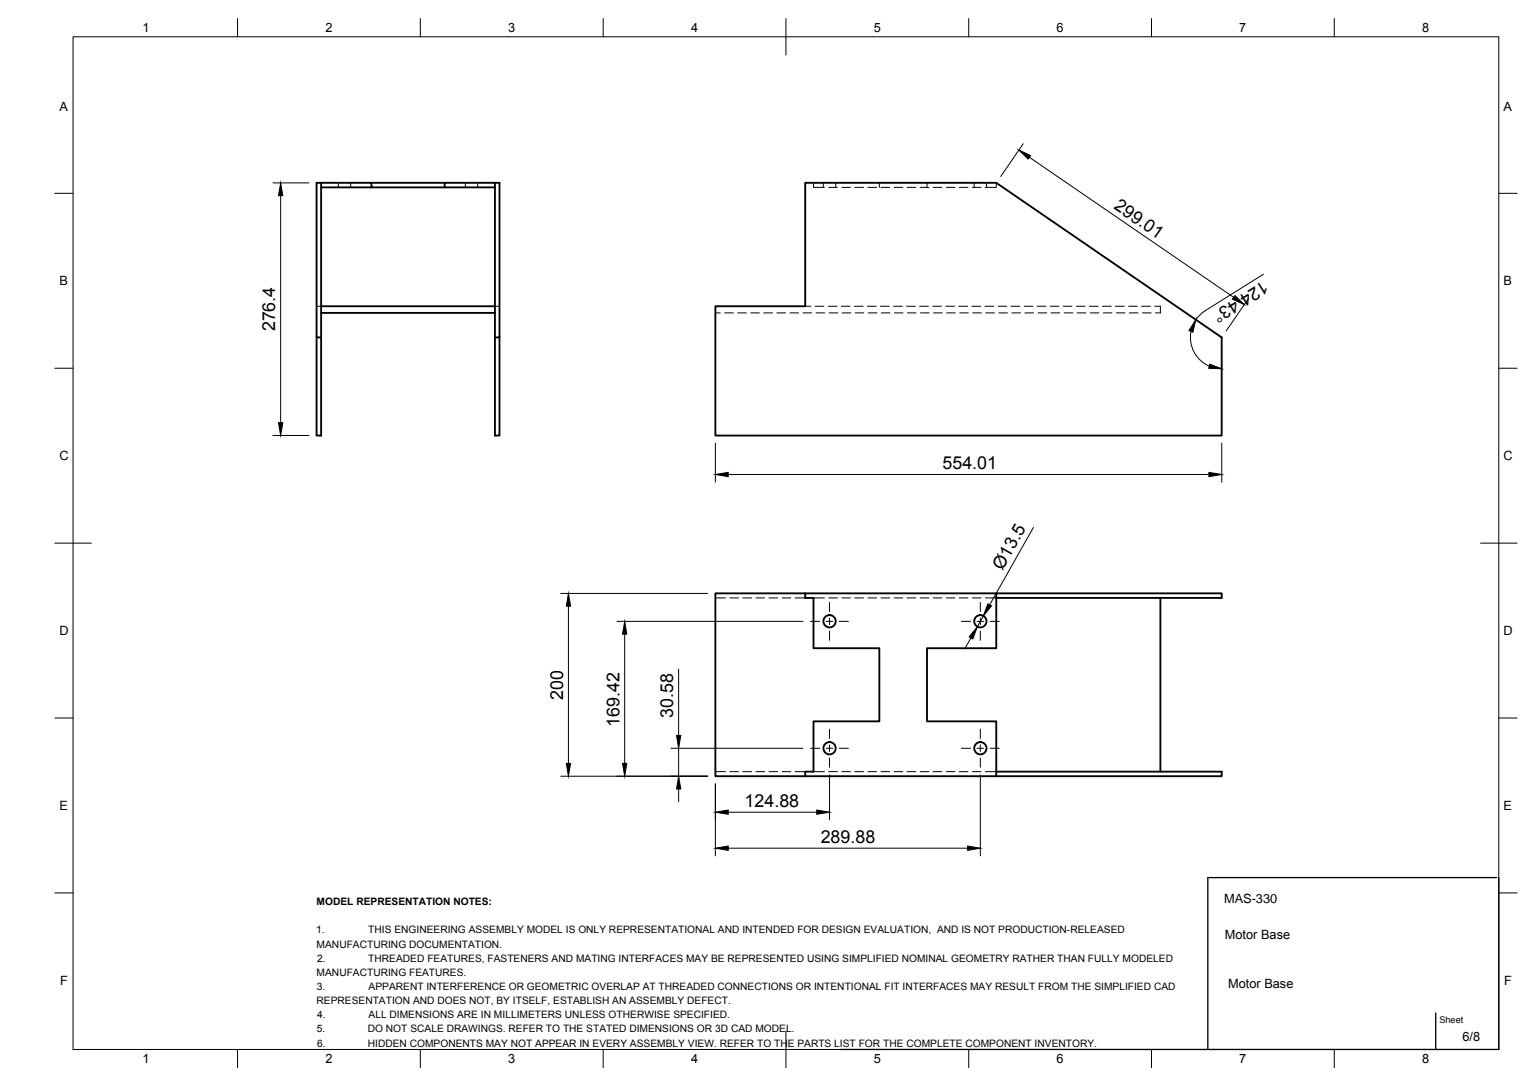
ISO-10303-21;
HEADER;
/* Generated by software containing ST-Developer
 * from STEP Tools, Inc. (www.steptools.com) 
 */

FILE_DESCRIPTION(
/* description */ ('STEP AP214'),
/* implementation_level */ '2;1');

FILE_NAME(
/* name */ 'Motor Base.step',
/* time_stamp */ '2026-10-12T14:05:15-07:00',
/* author */ (''),
/* organization */ (''),
/* preprocessor_version */ 'ST-DEVELOPER v20.2',
/* originating_system */ 'Autodesk Translation Framework v15.15.0.0',
/* authorisation */ '');

FILE_SCHEMA (('AUTOMOTIVE_DESIGN { 1 0 10303 214 3 1 1 }'));
ENDSEC;

DATA;
#10=MECHANICAL_DESIGN_GEOMETRIC_PRESENTATION_REPRESENTATION('',(#285),#39959);
#271=SHAPE_REPRESENTATION_RELATIONSHIP('SRR','None',#40005,#278);
#278=ADVANCED_BREP_SHAPE_REPRESENTATION('',(#293),#39955);
#285=STYLED_ITEM('',(#40046),#293);
#293=MANIFOLD_SOLID_BREP('Body1',#18262);
#391=PLANE('',#18765);
#392=PLANE('',#18766);
#393=PLANE('',#18767);
#394=PLANE('',#18768);
#395=PLANE('',#18769);
#396=PLANE('',#18770);
#397=PLANE('',#18771);
#398=PLANE('',#18772);
#399=PLANE('',#18773);
#400=PLANE('',#18774);
#401=PLANE('',#18775);
#402=PLANE('',#18776);
#403=PLANE('',#18777);
#404=PLANE('',#18778);
#405=PLANE('',#18779);
#406=PLANE('',#18780);
#407=PLANE('',#18781);
#408=PLANE('',#18782);
#409=PLANE('',#18783);
#410=PLANE('',#18784);
#411=PLANE('',#18785);
#412=PLANE('',#18786);
#413=PLANE('',#18787);
#414=PLANE('',#18788);
#415=PLANE('',#18789);
#416=PLANE('',#18790);
#417=PLANE('',#18791);
#418=PLANE('',#18792);
#956=FACE_BOUND('',#6112,.T.);
#957=FACE_BOUND('',#6113,.T.);
#958=FACE_BOUND('',#6114,.T.);
#959=FACE_BOUND('',#6115,.T.);
#960=FACE_BOUND('',#6117,.T.);
#961=FACE_BOUND('',#6118,.T.);
#962=FACE_BOUND('',#6119,.T.);
#963=FACE_BOUND('',#6120,.T.);
#1686=LINE('',#30305,#3259);
#1687=LINE('',#30311,#3260);
#1688=LINE('',#30317,#3261);
#1689=LINE('',#30323,#3262);
#1690=LINE('',#30328,#3263);
#1691=LINE('',#30330,#3264);
#1692=LINE('',#30332,#3265);
#1693=LINE('',#30334,#3266);
#1694=LINE('',#30336,#3267);
#1695=LINE('',#30338,#3268);
#1696=LINE('',#30340,#3269);
#1697=LINE('',#30342,#3270);
#1698=LINE('',#30344,#3271);
#1699=LINE('',#30346,#3272);
#1700=LINE('',#30348,#3273);
#1701=LINE('',#30349,#3274);
#1702=LINE('',#30353,#3275);
#1703=LINE('',#30355,#3276);
#1704=LINE('',#30357,#3277);
#1705=LINE('',#30359,#3278);
#1706=LINE('',#30361,#3279);
#1707=LINE('',#30363,#3280);
#1708=LINE('',#30365,#3281);
#1709=LINE('',#30367,#3282);
#1710=LINE('',#30369,#3283);
#1711=LINE('',#30371,#3284);
#1712=LINE('',#30373,#3285);
#1713=LINE('',#30374,#3286);
#1714=LINE('',#30377,#3287);
#1715=LINE('',#30379,#3288);
#1716=LINE('',#30380,#3289);
#1717=LINE('',#30383,#3290);
#1718=LINE('',#30385,#3291);
#1719=LINE('',#30386,#3292);
#1720=LINE('',#30389,#3293);
#1721=LINE('',#30391,#3294);
#1722=LINE('',#30392,#3295);
#1723=LINE('',#30395,#3296);
#1724=LINE('',#30397,#3297);
#1725=LINE('',#30398,#3298);
#1726=LINE('',#30400,#3299);
#1727=LINE('',#30401,#3300);
#1728=LINE('',#30404,#3301);
#1729=LINE('',#30406,#3302);
#1730=LINE('',#30407,#3303);
#1731=LINE('',#30410,#3304);
#1732=LINE('',#30412,#3305);
#1733=LINE('',#30413,#3306);
#1734=LINE('',#30416,#3307);
#1735=LINE('',#30418,#3308);
#1736=LINE('',#30419,#3309);
#1737=LINE('',#30422,#3310);
#1738=LINE('',#30424,#3311);
#1739=LINE('',#30425,#3312);
#1740=LINE('',#30427,#3313);
#1741=LINE('',#30428,#3314);
#1742=LINE('',#30432,#3315);
#1743=LINE('',#30434,#3316);
#1744=LINE('',#30435,#3317);
#1745=LINE('',#30437,#3318);
#1746=LINE('',#30439,#3319);
#1747=LINE('',#30440,#3320);
#1748=LINE('',#30443,#3321);
#1749=LINE('',#30444,#3322);
#1750=LINE('',#30447,#3323);
#1751=LINE('',#30448,#3324);
#1752=LINE('',#30450,#3325);
#1753=LINE('',#30452,#3326);
#1754=LINE('',#30454,#3327);
#1755=LINE('',#30456,#3328);
#1756=LINE('',#30457,#3329);
#1757=LINE('',#30460,#3330);
#1758=LINE('',#30461,#3331);
#1759=LINE('',#30462,#3332);
#1760=LINE('',#30464,#3333);
#1761=LINE('',#30465,#3334);
#1762=LINE('',#30468,#3335);
#1763=LINE('',#30469,#3336);
#1764=LINE('',#30471,#3337);
#1765=LINE('',#30475,#3338);
#1766=LINE('',#30476,#3339);
#1767=LINE('',#30479,#3340);
#1768=LINE('',#30480,#3341);
#1769=LINE('',#30482,#3342);
#1770=LINE('',#30484,#3343);
#1771=LINE('',#30487,#3344);
#3259=VECTOR('',#21100,6.75000000000001);
#3260=VECTOR('',#21107,6.74999999999998);
#3261=VECTOR('',#21114,6.74999999999998);
#3262=VECTOR('',#21121,6.75000000000001);
#3263=VECTOR('',#21126,1000.);
#3264=VECTOR('',#21127,1000.);
#3265=VECTOR('',#21128,1000.);
#3266=VECTOR('',#21129,1000.);
#3267=VECTOR('',#21130,1000.);
#3268=VECTOR('',#21131,1000.);
#3269=VECTOR('',#21132,1000.);
#3270=VECTOR('',#21133,1000.);
#3271=VECTOR('',#21134,1000.);
#3272=VECTOR('',#21135,1000.);
#3273=VECTOR('',#21136,1000.);
#3274=VECTOR('',#21137,1000.);
#3275=VECTOR('',#21140,1000.);
#3276=VECTOR('',#21141,1000.);
#3277=VECTOR('',#21142,1000.);
#3278=VECTOR('',#21143,1000.);
#3279=VECTOR('',#21144,1000.);
#3280=VECTOR('',#21145,1000.);
#3281=VECTOR('',#21146,1000.);
#3282=VECTOR('',#21147,1000.);
#3283=VECTOR('',#21148,1000.);
#3284=VECTOR('',#21149,1000.);
#3285=VECTOR('',#21150,1000.);
#3286=VECTOR('',#21151,1000.);
#3287=VECTOR('',#21154,1000.);
#3288=VECTOR('',#21155,1000.);
#3289=VECTOR('',#21156,1000.);
#3290=VECTOR('',#21159,1000.);
#3291=VECTOR('',#21160,1000.);
#3292=VECTOR('',#21161,1000.);
#3293=VECTOR('',#21164,1000.);
#3294=VECTOR('',#21165,1000.);
#3295=VECTOR('',#21166,1000.);
#3296=VECTOR('',#21169,1000.);
#3297=VECTOR('',#21170,1000.);
#3298=VECTOR('',#21171,1000.);
#3299=VECTOR('',#21174,1000.);
#3300=VECTOR('',#21175,1000.);
#3301=VECTOR('',#21178,1000.);
#3302=VECTOR('',#21179,1000.);
#3303=VECTOR('',#21180,1000.);
#3304=VECTOR('',#21183,1000.);
#3305=VECTOR('',#21184,1000.);
#3306=VECTOR('',#21185,1000.);
#3307=VECTOR('',#21188,1000.);
#3308=VECTOR('',#21189,1000.);
#3309=VECTOR('',#21190,1000.);
#3310=VECTOR('',#21193,1000.);
#3311=VECTOR('',#21194,1000.);
#3312=VECTOR('',#21195,1000.);
#3313=VECTOR('',#21198,1000.);
#3314=VECTOR('',#21199,1000.);
#3315=VECTOR('',#21204,1000.);
#3316=VECTOR('',#21205,1000.);
#3317=VECTOR('',#21206,1000.);
#3318=VECTOR('',#21207,1000.);
#3319=VECTOR('',#21208,1000.);
#3320=VECTOR('',#21209,1000.);
#3321=VECTOR('',#21212,1000.);
#3322=VECTOR('',#21213,1000.);
#3323=VECTOR('',#21216,1000.);
#3324=VECTOR('',#21217,1000.);
#3325=VECTOR('',#21220,1000.);
#3326=VECTOR('',#21221,1000.);
#3327=VECTOR('',#21222,1000.);
#3328=VECTOR('',#21223,1000.);
#3329=VECTOR('',#21224,1000.);
#3330=VECTOR('',#21227,1000.);
#3331=VECTOR('',#21228,1000.);
#3332=VECTOR('',#21229,1000.);
#3333=VECTOR('',#21230,1000.);
#3334=VECTOR('',#21231,1000.);
#3335=VECTOR('',#21234,1000.);
#3336=VECTOR('',#21235,1000.);
#3337=VECTOR('',#21238,1000.);
#3338=VECTOR('',#21243,1000.);
#3339=VECTOR('',#21244,1000.);
#3340=VECTOR('',#21247,1000.);
#3341=VECTOR('',#21248,1000.);
#3342=VECTOR('',#21251,1000.);
#3343=VECTOR('',#21254,1000.);
#3344=VECTOR('',#21259,1000.);
#4652=CYLINDRICAL_SURFACE('',#18753,6.75000000000001);
#4653=CYLINDRICAL_SURFACE('',#18756,6.74999999999998);
#4654=CYLINDRICAL_SURFACE('',#18759,6.74999999999998);
#4655=CYLINDRICAL_SURFACE('',#18762,6.75000000000001);
#5022=FACE_OUTER_BOUND('',#6095,.T.);
#5023=FACE_OUTER_BOUND('',#6096,.T.);
#5024=FACE_OUTER_BOUND('',#6097,.T.);
#5025=FACE_OUTER_BOUND('',#6098,.T.);
#5026=FACE_OUTER_BOUND('',#6099,.T.);
#5027=FACE_OUTER_BOUND('',#6100,.T.);
#5028=FACE_OUTER_BOUND('',#6101,.T.);
#5029=FACE_OUTER_BOUND('',#6102,.T.);
#5030=FACE_OUTER_BOUND('',#6103,.T.);
#5031=FACE_OUTER_BOUND('',#6104,.T.);
#5032=FACE_OUTER_BOUND('',#6105,.T.);
#5033=FACE_OUTER_BOUND('',#6106,.T.);
#5034=FACE_OUTER_BOUND('',#6107,.T.);
#5035=FACE_OUTER_BOUND('',#6108,.T.);
#5036=FACE_OUTER_BOUND('',#6109,.T.);
#5037=FACE_OUTER_BOUND('',#6110,.T.);
#5038=FACE_OUTER_BOUND('',#6111,.T.);
#5039=FACE_OUTER_BOUND('',#6116,.T.);
#5040=FACE_OUTER_BOUND('',#6121,.T.);
#5041=FACE_OUTER_BOUND('',#6122,.T.);
#5042=FACE_OUTER_BOUND('',#6123,.T.);
#5043=FACE_OUTER_BOUND('',#6124,.T.);
#5044=FACE_OUTER_BOUND('',#6125,.T.);
#5045=FACE_OUTER_BOUND('',#6126,.T.);
#5046=FACE_OUTER_BOUND('',#6127,.T.);
#5047=FACE_OUTER_BOUND('',#6128,.T.);
#5048=FACE_OUTER_BOUND('',#6129,.T.);
#5049=FACE_OUTER_BOUND('',#6130,.T.);
#5050=FACE_OUTER_BOUND('',#6131,.T.);
#5051=FACE_OUTER_BOUND('',#6132,.T.);
#5052=FACE_OUTER_BOUND('',#6133,.T.);
#5053=FACE_OUTER_BOUND('',#6134,.T.);
#6095=EDGE_LOOP('',(#13074,#13075,#13076,#13077));
#6096=EDGE_LOOP('',(#13078,#13079,#13080,#13081));
#6097=EDGE_LOOP('',(#13082,#13083,#13084,#13085));
#6098=EDGE_LOOP('',(#13086,#13087,#13088,#13089));
#6099=EDGE_LOOP('',(#13090,#13091,#13092,#13093,#13094,#13095,#13096,#13097,
#13098,#13099,#13100,#13101));
#6100=EDGE_LOOP('',(#13102,#13103,#13104,#13105,#13106,#13107,#13108,#13109,
#13110,#13111,#13112,#13113));
#6101=EDGE_LOOP('',(#13114,#13115,#13116,#13117));
#6102=EDGE_LOOP('',(#13118,#13119,#13120,#13121));
#6103=EDGE_LOOP('',(#13122,#13123,#13124,#13125));
#6104=EDGE_LOOP('',(#13126,#13127,#13128,#13129));
#6105=EDGE_LOOP('',(#13130,#13131,#13132,#13133));
#6106=EDGE_LOOP('',(#13134,#13135,#13136,#13137));
#6107=EDGE_LOOP('',(#13138,#13139,#13140,#13141));
#6108=EDGE_LOOP('',(#13142,#13143,#13144,#13145));
#6109=EDGE_LOOP('',(#13146,#13147,#13148,#13149));
#6110=EDGE_LOOP('',(#13150,#13151,#13152,#13153));
#6111=EDGE_LOOP('',(#13154,#13155,#13156,#13157,#13158,#13159,#13160,#13161,
#13162,#13163,#13164,#13165));
#6112=EDGE_LOOP('',(#13166));
#6113=EDGE_LOOP('',(#13167));
#6114=EDGE_LOOP('',(#13168));
#6115=EDGE_LOOP('',(#13169));
#6116=EDGE_LOOP('',(#13170,#13171,#13172,#13173,#13174,#13175,#13176,#13177,
#13178,#13179,#13180,#13181,#13182,#13183,#13184,#13185,#13186,#13187));
#6117=EDGE_LOOP('',(#13188));
#6118=EDGE_LOOP('',(#13189));
#6119=EDGE_LOOP('',(#13190));
#6120=EDGE_LOOP('',(#13191));
#6121=EDGE_LOOP('',(#13192,#13193,#13194,#13195));
#6122=EDGE_LOOP('',(#13196,#13197,#13198,#13199));
#6123=EDGE_LOOP('',(#13200,#13201,#13202,#13203,#13204,#13205,#13206,#13207));
#6124=EDGE_LOOP('',(#13208,#13209,#13210,#13211,#13212,#13213,#13214,#13215));
#6125=EDGE_LOOP('',(#13216,#13217,#13218,#13219));
#6126=EDGE_LOOP('',(#13220,#13221,#13222,#13223));
#6127=EDGE_LOOP('',(#13224,#13225,#13226,#13227,#13228,#13229,#13230));
#6128=EDGE_LOOP('',(#13231,#13232,#13233,#13234));
#6129=EDGE_LOOP('',(#13235,#13236,#13237,#13238));
#6130=EDGE_LOOP('',(#13239,#13240,#13241,#13242));
#6131=EDGE_LOOP('',(#13243,#13244,#13245,#13246));
#6132=EDGE_LOOP('',(#13247,#13248,#13249,#13250,#13251,#13252,#13253));
#6133=EDGE_LOOP('',(#13254,#13255,#13256,#13257));
#6134=EDGE_LOOP('',(#13258,#13259,#13260,#13261));
#7191=CIRCLE('',#18754,6.75000000000001);
#7192=CIRCLE('',#18755,6.75000000000001);
#7193=CIRCLE('',#18757,6.74999999999998);
#7194=CIRCLE('',#18758,6.74999999999998);
#7195=CIRCLE('',#18760,6.74999999999998);
#7196=CIRCLE('',#18761,6.74999999999998);
#7197=CIRCLE('',#18763,6.75000000000001);
#7198=CIRCLE('',#18764,6.75000000000001);
#8024=VERTEX_POINT('',#30302);
#8025=VERTEX_POINT('',#30304);
#8026=VERTEX_POINT('',#30308);
#8027=VERTEX_POINT('',#30310);
#8028=VERTEX_POINT('',#30314);
#8029=VERTEX_POINT('',#30316);
#8030=VERTEX_POINT('',#30320);
#8031=VERTEX_POINT('',#30322);
#8032=VERTEX_POINT('',#30326);
#8033=VERTEX_POINT('',#30327);
#8034=VERTEX_POINT('',#30329);
#8035=VERTEX_POINT('',#30331);
#8036=VERTEX_POINT('',#30333);
#8037=VERTEX_POINT('',#30335);
#8038=VERTEX_POINT('',#30337);
#8039=VERTEX_POINT('',#30339);
#8040=VERTEX_POINT('',#30341);
#8041=VERTEX_POINT('',#30343);
#8042=VERTEX_POINT('',#30345);
#8043=VERTEX_POINT('',#30347);
#8044=VERTEX_POINT('',#30351);
#8045=VERTEX_POINT('',#30352);
#8046=VERTEX_POINT('',#30354);
#8047=VERTEX_POINT('',#30356);
#8048=VERTEX_POINT('',#30358);
#8049=VERTEX_POINT('',#30360);
#8050=VERTEX_POINT('',#30362);
#8051=VERTEX_POINT('',#30364);
#8052=VERTEX_POINT('',#30366);
#8053=VERTEX_POINT('',#30368);
#8054=VERTEX_POINT('',#30370);
#8055=VERTEX_POINT('',#30372);
#8056=VERTEX_POINT('',#30376);
#8057=VERTEX_POINT('',#30378);
#8058=VERTEX_POINT('',#30382);
#8059=VERTEX_POINT('',#30384);
#8060=VERTEX_POINT('',#30388);
#8061=VERTEX_POINT('',#30390);
#8062=VERTEX_POINT('',#30394);
#8063=VERTEX_POINT('',#30396);
#8064=VERTEX_POINT('',#30403);
#8065=VERTEX_POINT('',#30405);
#8066=VERTEX_POINT('',#30409);
#8067=VERTEX_POINT('',#30411);
#8068=VERTEX_POINT('',#30415);
#8069=VERTEX_POINT('',#30417);
#8070=VERTEX_POINT('',#30421);
#8071=VERTEX_POINT('',#30423);
#8072=VERTEX_POINT('',#30431);
#8073=VERTEX_POINT('',#30433);
#8074=VERTEX_POINT('',#30436);
#8075=VERTEX_POINT('',#30438);
#8076=VERTEX_POINT('',#30442);
#8077=VERTEX_POINT('',#30446);
#8078=VERTEX_POINT('',#30451);
#8079=VERTEX_POINT('',#30453);
#8080=VERTEX_POINT('',#30455);
#8081=VERTEX_POINT('',#30459);
#8082=VERTEX_POINT('',#30463);
#8083=VERTEX_POINT('',#30467);
#8084=VERTEX_POINT('',#30474);
#8085=VERTEX_POINT('',#30478);
#9917=EDGE_CURVE('',#8024,#8024,#7191,.T.);
#9918=EDGE_CURVE('',#8024,#8025,#1686,.T.);
#9919=EDGE_CURVE('',#8025,#8025,#7192,.T.);
#9920=EDGE_CURVE('',#8026,#8026,#7193,.T.);
#9921=EDGE_CURVE('',#8026,#8027,#1687,.T.);
#9922=EDGE_CURVE('',#8027,#8027,#7194,.T.);
#9923=EDGE_CURVE('',#8028,#8028,#7195,.T.);
#9924=EDGE_CURVE('',#8028,#8029,#1688,.T.);
#9925=EDGE_CURVE('',#8029,#8029,#7196,.T.);
#9926=EDGE_CURVE('',#8030,#8030,#7197,.T.);
#9927=EDGE_CURVE('',#8030,#8031,#1689,.T.);
#9928=EDGE_CURVE('',#8031,#8031,#7198,.T.);
#9929=EDGE_CURVE('',#8032,#8033,#1690,.T.);
#9930=EDGE_CURVE('',#8034,#8032,#1691,.T.);
#9931=EDGE_CURVE('',#8035,#8034,#1692,.T.);
#9932=EDGE_CURVE('',#8036,#8035,#1693,.T.);
#9933=EDGE_CURVE('',#8037,#8036,#1694,.T.);
#9934=EDGE_CURVE('',#8038,#8037,#1695,.T.);
#9935=EDGE_CURVE('',#8039,#8038,#1696,.T.);
#9936=EDGE_CURVE('',#8039,#8040,#1697,.T.);
#9937=EDGE_CURVE('',#8040,#8041,#1698,.T.);
#9938=EDGE_CURVE('',#8042,#8041,#1699,.T.);
#9939=EDGE_CURVE('',#8043,#8042,#1700,.T.);
#9940=EDGE_CURVE('',#8033,#8043,#1701,.T.);
#9941=EDGE_CURVE('',#8044,#8045,#1702,.T.);
#9942=EDGE_CURVE('',#8046,#8044,#1703,.T.);
#9943=EDGE_CURVE('',#8046,#8047,#1704,.T.);
#9944=EDGE_CURVE('',#8047,#8048,#1705,.T.);
#9945=EDGE_CURVE('',#8048,#8049,#1706,.T.);
#9946=EDGE_CURVE('',#8049,#8050,#1707,.T.);
#9947=EDGE_CURVE('',#8051,#8050,#1708,.T.);
#9948=EDGE_CURVE('',#8051,#8052,#1709,.T.);
#9949=EDGE_CURVE('',#8052,#8053,#1710,.T.);
#9950=EDGE_CURVE('',#8053,#8054,#1711,.T.);
#9951=EDGE_CURVE('',#8054,#8055,#1712,.T.);
#9952=EDGE_CURVE('',#8045,#8055,#1713,.T.);
#9953=EDGE_CURVE('',#8056,#8038,#1714,.T.);
#9954=EDGE_CURVE('',#8057,#8056,#1715,.T.);
#9955=EDGE_CURVE('',#8057,#8039,#1716,.T.);
#9956=EDGE_CURVE('',#8058,#8056,#1717,.T.);
#9957=EDGE_CURVE('',#8059,#8058,#1718,.T.);
#9958=EDGE_CURVE('',#8059,#8057,#1719,.T.);
#9959=EDGE_CURVE('',#8060,#8058,#1720,.T.);
#9960=EDGE_CURVE('',#8061,#8060,#1721,.T.);
#9961=EDGE_CURVE('',#8061,#8059,#1722,.T.);
#9962=EDGE_CURVE('',#8062,#8060,#1723,.T.);
#9963=EDGE_CURVE('',#8063,#8062,#1724,.T.);
#9964=EDGE_CURVE('',#8063,#8061,#1725,.T.);
#9965=EDGE_CURVE('',#8053,#8062,#1726,.T.);
#9966=EDGE_CURVE('',#8052,#8063,#1727,.T.);
#9967=EDGE_CURVE('',#8064,#8050,#1728,.T.);
#9968=EDGE_CURVE('',#8065,#8064,#1729,.T.);
#9969=EDGE_CURVE('',#8065,#8051,#1730,.T.);
#9970=EDGE_CURVE('',#8066,#8064,#1731,.T.);
#9971=EDGE_CURVE('',#8067,#8066,#1732,.T.);
#9972=EDGE_CURVE('',#8067,#8065,#1733,.T.);
#9973=EDGE_CURVE('',#8068,#8066,#1734,.T.);
#9974=EDGE_CURVE('',#8069,#8068,#1735,.T.);
#9975=EDGE_CURVE('',#8069,#8067,#1736,.T.);
#9976=EDGE_CURVE('',#8070,#8068,#1737,.T.);
#9977=EDGE_CURVE('',#8071,#8070,#1738,.T.);
#9978=EDGE_CURVE('',#8071,#8069,#1739,.T.);
#9979=EDGE_CURVE('',#8041,#8070,#1740,.T.);
#9980=EDGE_CURVE('',#8040,#8071,#1741,.T.);
#9981=EDGE_CURVE('',#8072,#8037,#1742,.T.);
#9982=EDGE_CURVE('',#8073,#8072,#1743,.T.);
#9983=EDGE_CURVE('',#8073,#8041,#1744,.T.);
#9984=EDGE_CURVE('',#8074,#8050,#1745,.T.);
#9985=EDGE_CURVE('',#8074,#8075,#1746,.T.);
#9986=EDGE_CURVE('',#8075,#8054,#1747,.T.);
#9987=EDGE_CURVE('',#8076,#8073,#1748,.T.);
#9988=EDGE_CURVE('',#8076,#8042,#1749,.T.);
#9989=EDGE_CURVE('',#8077,#8036,#1750,.T.);
#9990=EDGE_CURVE('',#8072,#8077,#1751,.T.);
#9991=EDGE_CURVE('',#8045,#8035,#1752,.T.);
#9992=EDGE_CURVE('',#8078,#8055,#1753,.T.);
#9993=EDGE_CURVE('',#8078,#8079,#1754,.T.);
#9994=EDGE_CURVE('',#8080,#8079,#1755,.T.);
#9995=EDGE_CURVE('',#8077,#8080,#1756,.T.);
#9996=EDGE_CURVE('',#8079,#8081,#1757,.T.);
#9997=EDGE_CURVE('',#8081,#8047,#1758,.T.);
#9998=EDGE_CURVE('',#8046,#8032,#1759,.T.);
#9999=EDGE_CURVE('',#8082,#8033,#1760,.T.);
#10000=EDGE_CURVE('',#8080,#8082,#1761,.T.);
#10001=EDGE_CURVE('',#8083,#8043,#1762,.T.);
#10002=EDGE_CURVE('',#8082,#8083,#1763,.T.);
#10003=EDGE_CURVE('',#8083,#8076,#1764,.T.);
#10004=EDGE_CURVE('',#8084,#8049,#1765,.T.);
#10005=EDGE_CURVE('',#8084,#8074,#1766,.T.);
#10006=EDGE_CURVE('',#8085,#8048,#1767,.T.);
#10007=EDGE_CURVE('',#8085,#8084,#1768,.T.);
#10008=EDGE_CURVE('',#8081,#8085,#1769,.T.);
#10009=EDGE_CURVE('',#8075,#8078,#1770,.T.);
#10010=EDGE_CURVE('',#8044,#8034,#1771,.T.);
#13074=ORIENTED_EDGE('',*,*,#9917,.F.);
#13075=ORIENTED_EDGE('',*,*,#9918,.T.);
#13076=ORIENTED_EDGE('',*,*,#9919,.T.);
#13077=ORIENTED_EDGE('',*,*,#9918,.F.);
#13078=ORIENTED_EDGE('',*,*,#9920,.F.);
#13079=ORIENTED_EDGE('',*,*,#9921,.T.);
#13080=ORIENTED_EDGE('',*,*,#9922,.T.);
#13081=ORIENTED_EDGE('',*,*,#9921,.F.);
#13082=ORIENTED_EDGE('',*,*,#9923,.F.);
#13083=ORIENTED_EDGE('',*,*,#9924,.T.);
#13084=ORIENTED_EDGE('',*,*,#9925,.T.);
#13085=ORIENTED_EDGE('',*,*,#9924,.F.);
#13086=ORIENTED_EDGE('',*,*,#9926,.F.);
#13087=ORIENTED_EDGE('',*,*,#9927,.T.);
#13088=ORIENTED_EDGE('',*,*,#9928,.T.);
#13089=ORIENTED_EDGE('',*,*,#9927,.F.);
#13090=ORIENTED_EDGE('',*,*,#9929,.F.);
#13091=ORIENTED_EDGE('',*,*,#9930,.F.);
#13092=ORIENTED_EDGE('',*,*,#9931,.F.);
#13093=ORIENTED_EDGE('',*,*,#9932,.F.);
#13094=ORIENTED_EDGE('',*,*,#9933,.F.);
#13095=ORIENTED_EDGE('',*,*,#9934,.F.);
#13096=ORIENTED_EDGE('',*,*,#9935,.F.);
#13097=ORIENTED_EDGE('',*,*,#9936,.T.);
#13098=ORIENTED_EDGE('',*,*,#9937,.T.);
#13099=ORIENTED_EDGE('',*,*,#9938,.F.);
#13100=ORIENTED_EDGE('',*,*,#9939,.F.);
#13101=ORIENTED_EDGE('',*,*,#9940,.F.);
#13102=ORIENTED_EDGE('',*,*,#9941,.F.);
#13103=ORIENTED_EDGE('',*,*,#9942,.F.);
#13104=ORIENTED_EDGE('',*,*,#9943,.T.);
#13105=ORIENTED_EDGE('',*,*,#9944,.T.);
#13106=ORIENTED_EDGE('',*,*,#9945,.T.);
#13107=ORIENTED_EDGE('',*,*,#9946,.T.);
#13108=ORIENTED_EDGE('',*,*,#9947,.F.);
#13109=ORIENTED_EDGE('',*,*,#9948,.T.);
#13110=ORIENTED_EDGE('',*,*,#9949,.T.);
#13111=ORIENTED_EDGE('',*,*,#9950,.T.);
#13112=ORIENTED_EDGE('',*,*,#9951,.T.);
#13113=ORIENTED_EDGE('',*,*,#9952,.F.);
#13114=ORIENTED_EDGE('',*,*,#9953,.F.);
#13115=ORIENTED_EDGE('',*,*,#9954,.F.);
#13116=ORIENTED_EDGE('',*,*,#9955,.T.);
#13117=ORIENTED_EDGE('',*,*,#9935,.T.);
#13118=ORIENTED_EDGE('',*,*,#9956,.F.);
#13119=ORIENTED_EDGE('',*,*,#9957,.F.);
#13120=ORIENTED_EDGE('',*,*,#9958,.T.);
#13121=ORIENTED_EDGE('',*,*,#9954,.T.);
#13122=ORIENTED_EDGE('',*,*,#9959,.F.);
#13123=ORIENTED_EDGE('',*,*,#9960,.F.);
#13124=ORIENTED_EDGE('',*,*,#9961,.T.);
#13125=ORIENTED_EDGE('',*,*,#9957,.T.);
#13126=ORIENTED_EDGE('',*,*,#9962,.F.);
#13127=ORIENTED_EDGE('',*,*,#9963,.F.);
#13128=ORIENTED_EDGE('',*,*,#9964,.T.);
#13129=ORIENTED_EDGE('',*,*,#9960,.T.);
#13130=ORIENTED_EDGE('',*,*,#9965,.F.);
#13131=ORIENTED_EDGE('',*,*,#9949,.F.);
#13132=ORIENTED_EDGE('',*,*,#9966,.T.);
#13133=ORIENTED_EDGE('',*,*,#9963,.T.);
#13134=ORIENTED_EDGE('',*,*,#9967,.F.);
#13135=ORIENTED_EDGE('',*,*,#9968,.F.);
#13136=ORIENTED_EDGE('',*,*,#9969,.T.);
#13137=ORIENTED_EDGE('',*,*,#9947,.T.);
#13138=ORIENTED_EDGE('',*,*,#9970,.F.);
#13139=ORIENTED_EDGE('',*,*,#9971,.F.);
#13140=ORIENTED_EDGE('',*,*,#9972,.T.);
#13141=ORIENTED_EDGE('',*,*,#9968,.T.);
#13142=ORIENTED_EDGE('',*,*,#9973,.F.);
#13143=ORIENTED_EDGE('',*,*,#9974,.F.);
#13144=ORIENTED_EDGE('',*,*,#9975,.T.);
#13145=ORIENTED_EDGE('',*,*,#9971,.T.);
#13146=ORIENTED_EDGE('',*,*,#9976,.F.);
#13147=ORIENTED_EDGE('',*,*,#9977,.F.);
#13148=ORIENTED_EDGE('',*,*,#9978,.T.);
#13149=ORIENTED_EDGE('',*,*,#9974,.T.);
#13150=ORIENTED_EDGE('',*,*,#9979,.F.);
#13151=ORIENTED_EDGE('',*,*,#9937,.F.);
#13152=ORIENTED_EDGE('',*,*,#9980,.T.);
#13153=ORIENTED_EDGE('',*,*,#9977,.T.);
#13154=ORIENTED_EDGE('',*,*,#9936,.F.);
#13155=ORIENTED_EDGE('',*,*,#9955,.F.);
#13156=ORIENTED_EDGE('',*,*,#9958,.F.);
#13157=ORIENTED_EDGE('',*,*,#9961,.F.);
#13158=ORIENTED_EDGE('',*,*,#9964,.F.);
#13159=ORIENTED_EDGE('',*,*,#9966,.F.);
#13160=ORIENTED_EDGE('',*,*,#9948,.F.);
#13161=ORIENTED_EDGE('',*,*,#9969,.F.);
#13162=ORIENTED_EDGE('',*,*,#9972,.F.);
#13163=ORIENTED_EDGE('',*,*,#9975,.F.);
#13164=ORIENTED_EDGE('',*,*,#9978,.F.);
#13165=ORIENTED_EDGE('',*,*,#9980,.F.);
#13166=ORIENTED_EDGE('',*,*,#9917,.T.);
#13167=ORIENTED_EDGE('',*,*,#9920,.T.);
#13168=ORIENTED_EDGE('',*,*,#9923,.T.);
#13169=ORIENTED_EDGE('',*,*,#9926,.T.);
#13170=ORIENTED_EDGE('',*,*,#9953,.T.);
#13171=ORIENTED_EDGE('',*,*,#9934,.T.);
#13172=ORIENTED_EDGE('',*,*,#9981,.F.);
#13173=ORIENTED_EDGE('',*,*,#9982,.F.);
#13174=ORIENTED_EDGE('',*,*,#9983,.T.);
#13175=ORIENTED_EDGE('',*,*,#9979,.T.);
#13176=ORIENTED_EDGE('',*,*,#9976,.T.);
#13177=ORIENTED_EDGE('',*,*,#9973,.T.);
#13178=ORIENTED_EDGE('',*,*,#9970,.T.);
#13179=ORIENTED_EDGE('',*,*,#9967,.T.);
#13180=ORIENTED_EDGE('',*,*,#9984,.F.);
#13181=ORIENTED_EDGE('',*,*,#9985,.T.);
#13182=ORIENTED_EDGE('',*,*,#9986,.T.);
#13183=ORIENTED_EDGE('',*,*,#9950,.F.);
#13184=ORIENTED_EDGE('',*,*,#9965,.T.);
#13185=ORIENTED_EDGE('',*,*,#9962,.T.);
#13186=ORIENTED_EDGE('',*,*,#9959,.T.);
#13187=ORIENTED_EDGE('',*,*,#9956,.T.);
#13188=ORIENTED_EDGE('',*,*,#9919,.F.);
#13189=ORIENTED_EDGE('',*,*,#9922,.F.);
#13190=ORIENTED_EDGE('',*,*,#9925,.F.);
#13191=ORIENTED_EDGE('',*,*,#9928,.F.);
#13192=ORIENTED_EDGE('',*,*,#9938,.T.);
#13193=ORIENTED_EDGE('',*,*,#9983,.F.);
#13194=ORIENTED_EDGE('',*,*,#9987,.F.);
#13195=ORIENTED_EDGE('',*,*,#9988,.T.);
#13196=ORIENTED_EDGE('',*,*,#9933,.T.);
#13197=ORIENTED_EDGE('',*,*,#9989,.F.);
#13198=ORIENTED_EDGE('',*,*,#9990,.F.);
#13199=ORIENTED_EDGE('',*,*,#9981,.T.);
#13200=ORIENTED_EDGE('',*,*,#9989,.T.);
#13201=ORIENTED_EDGE('',*,*,#9932,.T.);
#13202=ORIENTED_EDGE('',*,*,#9991,.F.);
#13203=ORIENTED_EDGE('',*,*,#9952,.T.);
#13204=ORIENTED_EDGE('',*,*,#9992,.F.);
#13205=ORIENTED_EDGE('',*,*,#9993,.T.);
#13206=ORIENTED_EDGE('',*,*,#9994,.F.);
#13207=ORIENTED_EDGE('',*,*,#9995,.F.);
#13208=ORIENTED_EDGE('',*,*,#9994,.T.);
#13209=ORIENTED_EDGE('',*,*,#9996,.T.);
#13210=ORIENTED_EDGE('',*,*,#9997,.T.);
#13211=ORIENTED_EDGE('',*,*,#9943,.F.);
#13212=ORIENTED_EDGE('',*,*,#9998,.T.);
#13213=ORIENTED_EDGE('',*,*,#9929,.T.);
#13214=ORIENTED_EDGE('',*,*,#9999,.F.);
#13215=ORIENTED_EDGE('',*,*,#10000,.F.);
#13216=ORIENTED_EDGE('',*,*,#9940,.T.);
#13217=ORIENTED_EDGE('',*,*,#10001,.F.);
#13218=ORIENTED_EDGE('',*,*,#10002,.F.);
#13219=ORIENTED_EDGE('',*,*,#9999,.T.);
#13220=ORIENTED_EDGE('',*,*,#9939,.T.);
#13221=ORIENTED_EDGE('',*,*,#9988,.F.);
#13222=ORIENTED_EDGE('',*,*,#10003,.F.);
#13223=ORIENTED_EDGE('',*,*,#10001,.T.);
#13224=ORIENTED_EDGE('',*,*,#9987,.T.);
#13225=ORIENTED_EDGE('',*,*,#9982,.T.);
#13226=ORIENTED_EDGE('',*,*,#9990,.T.);
#13227=ORIENTED_EDGE('',*,*,#9995,.T.);
#13228=ORIENTED_EDGE('',*,*,#10000,.T.);
#13229=ORIENTED_EDGE('',*,*,#10002,.T.);
#13230=ORIENTED_EDGE('',*,*,#10003,.T.);
#13231=ORIENTED_EDGE('',*,*,#9946,.F.);
#13232=ORIENTED_EDGE('',*,*,#10004,.F.);
#13233=ORIENTED_EDGE('',*,*,#10005,.T.);
#13234=ORIENTED_EDGE('',*,*,#9984,.T.);
#13235=ORIENTED_EDGE('',*,*,#9945,.F.);
#13236=ORIENTED_EDGE('',*,*,#10006,.F.);
#13237=ORIENTED_EDGE('',*,*,#10007,.T.);
#13238=ORIENTED_EDGE('',*,*,#10004,.T.);
#13239=ORIENTED_EDGE('',*,*,#9944,.F.);
#13240=ORIENTED_EDGE('',*,*,#9997,.F.);
#13241=ORIENTED_EDGE('',*,*,#10008,.T.);
#13242=ORIENTED_EDGE('',*,*,#10006,.T.);
#13243=ORIENTED_EDGE('',*,*,#9951,.F.);
#13244=ORIENTED_EDGE('',*,*,#9986,.F.);
#13245=ORIENTED_EDGE('',*,*,#10009,.T.);
#13246=ORIENTED_EDGE('',*,*,#9992,.T.);
#13247=ORIENTED_EDGE('',*,*,#10005,.F.);
#13248=ORIENTED_EDGE('',*,*,#10007,.F.);
#13249=ORIENTED_EDGE('',*,*,#10008,.F.);
#13250=ORIENTED_EDGE('',*,*,#9996,.F.);
#13251=ORIENTED_EDGE('',*,*,#9993,.F.);
#13252=ORIENTED_EDGE('',*,*,#10009,.F.);
#13253=ORIENTED_EDGE('',*,*,#9985,.F.);
#13254=ORIENTED_EDGE('',*,*,#9998,.F.);
#13255=ORIENTED_EDGE('',*,*,#9942,.T.);
#13256=ORIENTED_EDGE('',*,*,#10010,.T.);
#13257=ORIENTED_EDGE('',*,*,#9930,.T.);
#13258=ORIENTED_EDGE('',*,*,#10010,.F.);
#13259=ORIENTED_EDGE('',*,*,#9941,.T.);
#13260=ORIENTED_EDGE('',*,*,#9991,.T.);
#13261=ORIENTED_EDGE('',*,*,#9931,.T.);
#17466=ADVANCED_FACE('',(#5022),#4652,.F.);
#17467=ADVANCED_FACE('',(#5023),#4653,.F.);
#17468=ADVANCED_FACE('',(#5024),#4654,.F.);
#17469=ADVANCED_FACE('',(#5025),#4655,.F.);
#17470=ADVANCED_FACE('',(#5026),#391,.T.);
#17471=ADVANCED_FACE('',(#5027),#392,.T.);
#17472=ADVANCED_FACE('',(#5028),#393,.T.);
#17473=ADVANCED_FACE('',(#5029),#394,.T.);
#17474=ADVANCED_FACE('',(#5030),#395,.T.);
#17475=ADVANCED_FACE('',(#5031),#396,.T.);
#17476=ADVANCED_FACE('',(#5032),#397,.T.);
#17477=ADVANCED_FACE('',(#5033),#398,.T.);
#17478=ADVANCED_FACE('',(#5034),#399,.T.);
#17479=ADVANCED_FACE('',(#5035),#400,.T.);
#17480=ADVANCED_FACE('',(#5036),#401,.T.);
#17481=ADVANCED_FACE('',(#5037),#402,.T.);
#17482=ADVANCED_FACE('',(#5038,#956,#957,#958,#959),#403,.F.);
#17483=ADVANCED_FACE('',(#5039,#960,#961,#962,#963),#404,.T.);
#17484=ADVANCED_FACE('',(#5040),#405,.F.);
#17485=ADVANCED_FACE('',(#5041),#406,.F.);
#17486=ADVANCED_FACE('',(#5042),#407,.F.);
#17487=ADVANCED_FACE('',(#5043),#408,.F.);
#17488=ADVANCED_FACE('',(#5044),#409,.F.);
#17489=ADVANCED_FACE('',(#5045),#410,.F.);
#17490=ADVANCED_FACE('',(#5046),#411,.F.);
#17491=ADVANCED_FACE('',(#5047),#412,.T.);
#17492=ADVANCED_FACE('',(#5048),#413,.T.);
#17493=ADVANCED_FACE('',(#5049),#414,.T.);
#17494=ADVANCED_FACE('',(#5050),#415,.T.);
#17495=ADVANCED_FACE('',(#5051),#416,.F.);
#17496=ADVANCED_FACE('',(#5052),#417,.F.);
#17497=ADVANCED_FACE('',(#5053),#418,.F.);
#18262=CLOSED_SHELL('',(#17466,#17467,#17468,#17469,#17470,#17471,#17472,
#17473,#17474,#17475,#17476,#17477,#17478,#17479,#17480,#17481,#17482,#17483,
#17484,#17485,#17486,#17487,#17488,#17489,#17490,#17491,#17492,#17493,#17494,
#17495,#17496,#17497));
#18752=AXIS2_PLACEMENT_3D('',#30300,#21094,#21095);
#18753=AXIS2_PLACEMENT_3D('',#30301,#21096,#21097);
#18754=AXIS2_PLACEMENT_3D('',#30303,#21098,#21099);
#18755=AXIS2_PLACEMENT_3D('',#30306,#21101,#21102);
#18756=AXIS2_PLACEMENT_3D('',#30307,#21103,#21104);
#18757=AXIS2_PLACEMENT_3D('',#30309,#21105,#21106);
#18758=AXIS2_PLACEMENT_3D('',#30312,#21108,#21109);
#18759=AXIS2_PLACEMENT_3D('',#30313,#21110,#21111);
#18760=AXIS2_PLACEMENT_3D('',#30315,#21112,#21113);
#18761=AXIS2_PLACEMENT_3D('',#30318,#21115,#21116);
#18762=AXIS2_PLACEMENT_3D('',#30319,#21117,#21118);
#18763=AXIS2_PLACEMENT_3D('',#30321,#21119,#21120);
#18764=AXIS2_PLACEMENT_3D('',#30324,#21122,#21123);
#18765=AXIS2_PLACEMENT_3D('',#30325,#21124,#21125);
#18766=AXIS2_PLACEMENT_3D('',#30350,#21138,#21139);
#18767=AXIS2_PLACEMENT_3D('',#30375,#21152,#21153);
#18768=AXIS2_PLACEMENT_3D('',#30381,#21157,#21158);
#18769=AXIS2_PLACEMENT_3D('',#30387,#21162,#21163);
#18770=AXIS2_PLACEMENT_3D('',#30393,#21167,#21168);
#18771=AXIS2_PLACEMENT_3D('',#30399,#21172,#21173);
#18772=AXIS2_PLACEMENT_3D('',#30402,#21176,#21177);
#18773=AXIS2_PLACEMENT_3D('',#30408,#21181,#21182);
#18774=AXIS2_PLACEMENT_3D('',#30414,#21186,#21187);
#18775=AXIS2_PLACEMENT_3D('',#30420,#21191,#21192);
#18776=AXIS2_PLACEMENT_3D('',#30426,#21196,#21197);
#18777=AXIS2_PLACEMENT_3D('',#30429,#21200,#21201);
#18778=AXIS2_PLACEMENT_3D('',#30430,#21202,#21203);
#18779=AXIS2_PLACEMENT_3D('',#30441,#21210,#21211);
#18780=AXIS2_PLACEMENT_3D('',#30445,#21214,#21215);
#18781=AXIS2_PLACEMENT_3D('',#30449,#21218,#21219);
#18782=AXIS2_PLACEMENT_3D('',#30458,#21225,#21226);
#18783=AXIS2_PLACEMENT_3D('',#30466,#21232,#21233);
#18784=AXIS2_PLACEMENT_3D('',#30470,#21236,#21237);
#18785=AXIS2_PLACEMENT_3D('',#30472,#21239,#21240);
#18786=AXIS2_PLACEMENT_3D('',#30473,#21241,#21242);
#18787=AXIS2_PLACEMENT_3D('',#30477,#21245,#21246);
#18788=AXIS2_PLACEMENT_3D('',#30481,#21249,#21250);
#18789=AXIS2_PLACEMENT_3D('',#30483,#21252,#21253);
#18790=AXIS2_PLACEMENT_3D('',#30485,#21255,#21256);
#18791=AXIS2_PLACEMENT_3D('',#30486,#21257,#21258);
#18792=AXIS2_PLACEMENT_3D('',#30488,#21260,#21261);
#21094=DIRECTION('axis',(0.,0.,1.));
#21095=DIRECTION('refdir',(1.,0.,0.));
#21096=DIRECTION('center_axis',(0.,1.,0.));
#21097=DIRECTION('ref_axis',(0.,0.,1.));
#21098=DIRECTION('center_axis',(0.,1.,0.));
#21099=DIRECTION('ref_axis',(0.,0.,-1.));
#21100=DIRECTION('',(0.,1.,0.));
#21101=DIRECTION('center_axis',(0.,1.,0.));
#21102=DIRECTION('ref_axis',(0.,0.,-1.));
#21103=DIRECTION('center_axis',(0.,1.,0.));
#21104=DIRECTION('ref_axis',(0.,0.,1.));
#21105=DIRECTION('center_axis',(0.,1.,0.));
#21106=DIRECTION('ref_axis',(0.,0.,-1.));
#21107=DIRECTION('',(0.,1.,0.));
#21108=DIRECTION('center_axis',(0.,1.,0.));
#21109=DIRECTION('ref_axis',(0.,0.,-1.));
#21110=DIRECTION('center_axis',(0.,1.,0.));
#21111=DIRECTION('ref_axis',(0.,0.,1.));
#21112=DIRECTION('center_axis',(0.,1.,0.));
#21113=DIRECTION('ref_axis',(0.,0.,1.));
#21114=DIRECTION('',(0.,1.,0.));
#21115=DIRECTION('center_axis',(0.,1.,0.));
#21116=DIRECTION('ref_axis',(0.,0.,1.));
#21117=DIRECTION('center_axis',(0.,1.,0.));
#21118=DIRECTION('ref_axis',(0.,0.,1.));
#21119=DIRECTION('center_axis',(0.,1.,0.));
#21120=DIRECTION('ref_axis',(0.,0.,1.));
#21121=DIRECTION('',(0.,1.,0.));
#21122=DIRECTION('center_axis',(0.,1.,0.));
#21123=DIRECTION('ref_axis',(0.,0.,1.));
#21124=DIRECTION('center_axis',(-1.,0.,-1.12538885307499E-16));
#21125=DIRECTION('ref_axis',(-1.12538885307499E-16,0.,1.));
#21126=DIRECTION('',(0.,-1.,0.));
#21127=DIRECTION('',(-1.14004428052113E-16,0.,1.));
#21128=DIRECTION('',(0.,-1.,0.));
#21129=DIRECTION('',(1.14004428052113E-16,0.,-1.));
#21130=DIRECTION('',(0.,-1.,0.));
#21131=DIRECTION('',(-1.32743918944454E-16,0.,1.));
#21132=DIRECTION('',(0.,1.,0.));
#21133=DIRECTION('',(1.38777878078144E-16,0.,-1.));
#21134=DIRECTION('',(0.,1.,0.));
#21135=DIRECTION('',(-9.28250249804007E-17,0.565386313251385,0.824826234299083));
#21136=DIRECTION('',(0.,1.,0.));
#21137=DIRECTION('',(1.25247756392721E-16,0.,-1.));
#21138=DIRECTION('center_axis',(1.,0.,-1.12538885307499E-16));
#21139=DIRECTION('ref_axis',(1.12538885307499E-16,0.,1.));
#21140=DIRECTION('',(0.,1.,0.));
#21141=DIRECTION('',(-1.12538885307499E-16,0.,-1.));
#21142=DIRECTION('',(0.,-1.,0.));
#21143=DIRECTION('',(-1.25247756392721E-16,0.,-1.));
#21144=DIRECTION('',(0.,1.,0.));
#21145=DIRECTION('',(9.28250249804007E-17,0.565386313251385,0.824826234299083));
#21146=DIRECTION('',(0.,1.,0.));
#21147=DIRECTION('',(1.38777878078144E-16,0.,1.));
#21148=DIRECTION('',(0.,1.,0.));
#21149=DIRECTION('',(1.32743918944454E-16,0.,1.));
#21150=DIRECTION('',(0.,-1.,0.));
#21151=DIRECTION('',(1.12538885307499E-16,0.,1.));
#21152=DIRECTION('center_axis',(0.,0.,1.));
#21153=DIRECTION('ref_axis',(1.,0.,0.));
#21154=DIRECTION('',(1.,0.,0.));
#21155=DIRECTION('',(0.,1.,0.));
#21156=DIRECTION('',(1.,0.,0.));
#21157=DIRECTION('center_axis',(-1.,0.,9.63735264431558E-17));
#21158=DIRECTION('ref_axis',(9.63735264431558E-17,0.,1.));
#21159=DIRECTION('',(9.63735264431558E-17,0.,1.));
#21160=DIRECTION('',(0.,1.,0.));
#21161=DIRECTION('',(9.63735264431558E-17,0.,1.));
#21162=DIRECTION('center_axis',(0.,0.,1.));
#21163=DIRECTION('ref_axis',(1.,0.,0.));
#21164=DIRECTION('',(1.,0.,0.));
#21165=DIRECTION('',(0.,1.,0.));
#21166=DIRECTION('',(1.,0.,0.));
#21167=DIRECTION('center_axis',(1.,0.,0.));
#21168=DIRECTION('ref_axis',(0.,0.,-1.));
#21169=DIRECTION('',(0.,0.,-1.));
#21170=DIRECTION('',(0.,1.,0.));
#21171=DIRECTION('',(0.,0.,-1.));
#21172=DIRECTION('center_axis',(0.,0.,1.));
#21173=DIRECTION('ref_axis',(1.,0.,0.));
#21174=DIRECTION('',(1.,0.,0.));
#21175=DIRECTION('',(1.,0.,0.));
#21176=DIRECTION('center_axis',(0.,0.,-1.));
#21177=DIRECTION('ref_axis',(-1.,0.,0.));
#21178=DIRECTION('',(-1.,0.,0.));
#21179=DIRECTION('',(0.,1.,0.));
#21180=DIRECTION('',(-1.,0.,0.));
#21181=DIRECTION('center_axis',(1.,0.,0.));
#21182=DIRECTION('ref_axis',(0.,0.,-1.));
#21183=DIRECTION('',(0.,0.,-1.));
#21184=DIRECTION('',(0.,1.,0.));
#21185=DIRECTION('',(0.,0.,-1.));
#21186=DIRECTION('center_axis',(0.,0.,-1.));
#21187=DIRECTION('ref_axis',(-1.,0.,0.));
#21188=DIRECTION('',(-1.,0.,0.));
#21189=DIRECTION('',(0.,1.,0.));
#21190=DIRECTION('',(-1.,0.,0.));
#21191=DIRECTION('center_axis',(-1.,0.,0.));
#21192=DIRECTION('ref_axis',(0.,0.,1.));
#21193=DIRECTION('',(0.,0.,1.));
#21194=DIRECTION('',(0.,1.,0.));
#21195=DIRECTION('',(0.,0.,1.));
#21196=DIRECTION('center_axis',(0.,0.,-1.));
#21197=DIRECTION('ref_axis',(-1.,0.,0.));
#21198=DIRECTION('',(-1.,0.,0.));
#21199=DIRECTION('',(-1.,0.,0.));
#21200=DIRECTION('center_axis',(0.,1.,0.));
#21201=DIRECTION('ref_axis',(0.,0.,1.));
#21202=DIRECTION('center_axis',(0.,1.,0.));
#21203=DIRECTION('ref_axis',(0.,0.,1.));
#21204=DIRECTION('',(-1.,0.,-1.38777878078144E-16));
#21205=DIRECTION('',(-1.32743918944454E-16,0.,1.));
#21206=DIRECTION('',(-1.,0.,-1.38777878078144E-16));
#21207=DIRECTION('',(1.,0.,-1.38777878078144E-16));
#21208=DIRECTION('',(1.32743918944454E-16,0.,1.));
#21209=DIRECTION('',(1.,0.,-1.38777878078144E-16));
#21210=DIRECTION('center_axis',(-7.84631128474524E-17,-0.824826234299083,
0.565386313251385));
#21211=DIRECTION('ref_axis',(-6.77673776348631E-34,-0.565386313251385,-0.824826234299084));
#21212=DIRECTION('',(-9.28250249804007E-17,0.565386313251385,0.824826234299083));
#21213=DIRECTION('',(-1.,0.,-1.38777878078144E-16));
#21214=DIRECTION('center_axis',(1.38777878078144E-16,0.,-1.));
#21215=DIRECTION('ref_axis',(-1.,0.,-1.38777878078145E-16));
#21216=DIRECTION('',(-1.,0.,-1.38777878078144E-16));
#21217=DIRECTION('',(0.,-1.,0.));
#21218=DIRECTION('center_axis',(0.,-1.,0.));
#21219=DIRECTION('ref_axis',(0.,0.,-1.));
#21220=DIRECTION('',(1.,0.,1.32222068111359E-16));
#21221=DIRECTION('',(1.,0.,-1.38777878078144E-16));
#21222=DIRECTION('',(1.41190366869118E-16,0.,1.));
#21223=DIRECTION('',(-1.,0.,-1.38777878078144E-16));
#21224=DIRECTION('',(-1.41190366869118E-16,0.,1.));
#21225=DIRECTION('center_axis',(1.38777878078144E-16,0.,-1.));
#21226=DIRECTION('ref_axis',(-1.,0.,-1.38777878078145E-16));
#21227=DIRECTION('',(0.,-1.,0.));
#21228=DIRECTION('',(1.,0.,-1.38777878078144E-16));
#21229=DIRECTION('',(1.,0.,1.32222068111359E-16));
#21230=DIRECTION('',(-1.,0.,-1.38777878078144E-16));
#21231=DIRECTION('',(0.,-1.,0.));
#21232=DIRECTION('center_axis',(0.,1.,0.));
#21233=DIRECTION('ref_axis',(0.,0.,1.));
#21234=DIRECTION('',(-1.,0.,-1.38777878078144E-16));
#21235=DIRECTION('',(1.25247756392721E-16,0.,-1.));
#21236=DIRECTION('center_axis',(-1.38777878078144E-16,0.,1.));
#21237=DIRECTION('ref_axis',(1.,0.,1.38777878078145E-16));
#21238=DIRECTION('',(0.,1.,0.));
#21239=DIRECTION('center_axis',(-1.,0.,-1.12538885307499E-16));
#21240=DIRECTION('ref_axis',(-1.12538885307499E-16,0.,1.));
#21241=DIRECTION('center_axis',(-7.84631128474524E-17,0.824826234299083,
-0.565386313251385));
#21242=DIRECTION('ref_axis',(-6.77673776348631E-34,0.565386313251385,0.824826234299084));
#21243=DIRECTION('',(1.,0.,-1.38777878078144E-16));
#21244=DIRECTION('',(9.28250249804007E-17,0.565386313251385,0.824826234299083));
#21245=DIRECTION('center_axis',(-1.38777878078144E-16,0.,-1.));
#21246=DIRECTION('ref_axis',(-1.,0.,1.38777878078145E-16));
#21247=DIRECTION('',(1.,0.,-1.38777878078144E-16));
#21248=DIRECTION('',(0.,1.,0.));
#21249=DIRECTION('center_axis',(0.,-1.,0.));
#21250=DIRECTION('ref_axis',(0.,0.,-1.));
#21251=DIRECTION('',(-1.25247756392721E-16,0.,-1.));
#21252=DIRECTION('center_axis',(1.38777878078144E-16,0.,1.));
#21253=DIRECTION('ref_axis',(1.,0.,-1.38777878078145E-16));
#21254=DIRECTION('',(0.,-1.,0.));
#21255=DIRECTION('center_axis',(1.,0.,-1.12538885307499E-16));
#21256=DIRECTION('ref_axis',(1.12538885307499E-16,0.,1.));
#21257=DIRECTION('center_axis',(0.,1.,0.));
#21258=DIRECTION('ref_axis',(0.,0.,1.));
#21259=DIRECTION('',(1.,0.,1.32222068111359E-16));
#21260=DIRECTION('center_axis',(-1.32222068111359E-16,0.,1.));
#21261=DIRECTION('ref_axis',(1.,0.,1.32222068111359E-16));
#30300=CARTESIAN_POINT('',(0.,0.,0.));
#30301=CARTESIAN_POINT('Origin',(-69.4209305758952,-120.,-82.5));
#30302=CARTESIAN_POINT('',(-69.4209305758952,-120.,-89.25));
#30303=CARTESIAN_POINT('Origin',(-69.4209305758952,-120.,-82.5));
#30304=CARTESIAN_POINT('',(-69.4209305758952,-115.,-89.25));
#30305=CARTESIAN_POINT('',(-69.4209305758952,-120.,-89.25));
#30306=CARTESIAN_POINT('Origin',(-69.4209305758952,-115.,-82.5));
#30307=CARTESIAN_POINT('Origin',(-69.4209305758952,-120.,-247.5));
#30308=CARTESIAN_POINT('',(-69.4209305758952,-120.,-254.25));
#30309=CARTESIAN_POINT('Origin',(-69.4209305758952,-120.,-247.5));
#30310=CARTESIAN_POINT('',(-69.4209305758952,-115.,-254.25));
#30311=CARTESIAN_POINT('',(-69.4209305758952,-120.,-254.25));
#30312=CARTESIAN_POINT('Origin',(-69.4209305758952,-115.,-247.5));
#30313=CARTESIAN_POINT('Origin',(69.4209305758952,-120.,-247.5));
#30314=CARTESIAN_POINT('',(69.4209305758952,-120.,-254.25));
#30315=CARTESIAN_POINT('Origin',(69.4209305758952,-120.,-247.5));
#30316=CARTESIAN_POINT('',(69.4209305758952,-115.,-254.25));
#30317=CARTESIAN_POINT('',(69.4209305758952,-120.,-254.25));
#30318=CARTESIAN_POINT('Origin',(69.4209305758952,-115.,-247.5));
#30319=CARTESIAN_POINT('Origin',(69.4209305758952,-120.,-82.5));
#30320=CARTESIAN_POINT('',(69.4209305758952,-120.,-89.25));
#30321=CARTESIAN_POINT('Origin',(69.4209305758952,-120.,-82.5));
#30322=CARTESIAN_POINT('',(69.4209305758952,-115.,-89.25));
#30323=CARTESIAN_POINT('',(69.4209305758952,-120.,-89.25));
#30324=CARTESIAN_POINT('Origin',(69.4209305758952,-115.,-82.5));
#30325=CARTESIAN_POINT('Origin',(95.,0.,1.06911941042124E-14));
#30326=CARTESIAN_POINT('',(95.,-257.272114237069,42.3824489701997));
#30327=CARTESIAN_POINT('',(95.,-391.404841890133,42.3824489701997));
#30328=CARTESIAN_POINT('',(95.,-250.,42.3824489701997));
#30329=CARTESIAN_POINT('',(95.0000000000001,-257.272114237069,-444.538560851304));
#30330=CARTESIAN_POINT('',(95.,-257.272114237069,42.3824489701998));
#30331=CARTESIAN_POINT('',(95.0000000000001,-250.,-444.538560851304));
#30332=CARTESIAN_POINT('',(95.0000000000001,-250.,-444.538560851304));
#30333=CARTESIAN_POINT('',(95.,-250.,-55.9088729914395));
#30334=CARTESIAN_POINT('',(95.,-250.,42.3824489701998));
#30335=CARTESIAN_POINT('',(95.,-115.,-55.9088729914395));
#30336=CARTESIAN_POINT('',(95.,-250.,-55.9088729914395));
#30337=CARTESIAN_POINT('',(95.,-115.,-65.));
#30338=CARTESIAN_POINT('',(95.,-115.,-55.9088729914395));
#30339=CARTESIAN_POINT('',(95.,-120.,-65.));
#30340=CARTESIAN_POINT('',(95.,-120.,-65.));
#30341=CARTESIAN_POINT('',(95.,-120.,-265.));
#30342=CARTESIAN_POINT('',(95.,-120.,-65.));
#30343=CARTESIAN_POINT('',(95.,-115.,-265.));
#30344=CARTESIAN_POINT('',(95.,-120.,-265.));
#30345=CARTESIAN_POINT('',(95.0000000000001,-284.055947712418,-511.630980392157));
#30346=CARTESIAN_POINT('',(95.0000000000001,-284.055947712418,-511.630980392157));
#30347=CARTESIAN_POINT('',(95.0000000000001,-391.404841890133,-511.630980392157));
#30348=CARTESIAN_POINT('',(95.0000000000001,-391.404841890133,-511.630980392157));
#30349=CARTESIAN_POINT('',(95.,-391.404841890133,42.3824489701997));
#30350=CARTESIAN_POINT('Origin',(-95.,0.,1.06911941042124E-14));
#30351=CARTESIAN_POINT('',(-95.0000000000001,-257.272114237069,-444.538560851304));
#30352=CARTESIAN_POINT('',(-95.0000000000001,-250.,-444.538560851304));
#30353=CARTESIAN_POINT('',(-95.,-250.,-444.538560851304));
#30354=CARTESIAN_POINT('',(-95.,-257.272114237069,42.3824489701997));
#30355=CARTESIAN_POINT('',(-95.,-257.272114237069,42.3824489701996));
#30356=CARTESIAN_POINT('',(-95.,-391.404841890133,42.3824489701997));
#30357=CARTESIAN_POINT('',(-95.,-250.,42.3824489701997));
#30358=CARTESIAN_POINT('',(-95.0000000000001,-391.404841890133,-511.630980392157));
#30359=CARTESIAN_POINT('',(-95.,-391.404841890133,42.3824489701997));
#30360=CARTESIAN_POINT('',(-95.0000000000001,-284.055947712418,-511.630980392157));
#30361=CARTESIAN_POINT('',(-95.0000000000001,-391.404841890133,-511.630980392157));
#30362=CARTESIAN_POINT('',(-95.,-115.,-265.));
#30363=CARTESIAN_POINT('',(-95.0000000000001,-284.055947712418,-511.630980392157));
#30364=CARTESIAN_POINT('',(-95.,-120.,-265.));
#30365=CARTESIAN_POINT('',(-95.,-120.,-265.));
#30366=CARTESIAN_POINT('',(-95.,-120.,-65.));
#30367=CARTESIAN_POINT('',(-95.,-120.,-265.));
#30368=CARTESIAN_POINT('',(-95.,-115.,-65.));
#30369=CARTESIAN_POINT('',(-95.,-120.,-65.));
#30370=CARTESIAN_POINT('',(-95.,-115.,-55.9088729914395));
#30371=CARTESIAN_POINT('',(-95.,-115.,-55.9088729914395));
#30372=CARTESIAN_POINT('',(-95.,-250.,-55.9088729914395));
#30373=CARTESIAN_POINT('',(-95.,-250.,-55.9088729914395));
#30374=CARTESIAN_POINT('',(-95.,-250.,42.3824489701996));
#30375=CARTESIAN_POINT('Origin',(39.9999999999999,-120.,-65.));
#30376=CARTESIAN_POINT('',(39.9999999999999,-115.,-65.));
#30377=CARTESIAN_POINT('',(39.9999999999999,-115.,-65.));
#30378=CARTESIAN_POINT('',(39.9999999999999,-120.,-65.));
#30379=CARTESIAN_POINT('',(39.9999999999999,-120.,-65.));
#30380=CARTESIAN_POINT('',(39.9999999999999,-120.,-65.));
#30381=CARTESIAN_POINT('Origin',(39.9999999999999,-120.,-137.));
#30382=CARTESIAN_POINT('',(39.9999999999999,-115.,-137.));
#30383=CARTESIAN_POINT('',(39.9999999999999,-115.,-137.));
#30384=CARTESIAN_POINT('',(39.9999999999999,-120.,-137.));
#30385=CARTESIAN_POINT('',(39.9999999999999,-120.,-137.));
#30386=CARTESIAN_POINT('',(39.9999999999999,-120.,-137.));
#30387=CARTESIAN_POINT('Origin',(-40.0000000000001,-120.,-137.));
#30388=CARTESIAN_POINT('',(-40.0000000000001,-115.,-137.));
#30389=CARTESIAN_POINT('',(-40.0000000000001,-115.,-137.));
#30390=CARTESIAN_POINT('',(-40.0000000000001,-120.,-137.));
#30391=CARTESIAN_POINT('',(-40.0000000000001,-120.,-137.));
#30392=CARTESIAN_POINT('',(-40.0000000000001,-120.,-137.));
#30393=CARTESIAN_POINT('Origin',(-40.0000000000001,-120.,-65.));
#30394=CARTESIAN_POINT('',(-40.0000000000001,-115.,-65.));
#30395=CARTESIAN_POINT('',(-40.0000000000001,-115.,-65.));
#30396=CARTESIAN_POINT('',(-40.0000000000001,-120.,-65.));
#30397=CARTESIAN_POINT('',(-40.0000000000001,-120.,-65.));
#30398=CARTESIAN_POINT('',(-40.0000000000001,-120.,-65.));
#30399=CARTESIAN_POINT('Origin',(-95.,-120.,-65.));
#30400=CARTESIAN_POINT('',(-95.,-115.,-65.));
#30401=CARTESIAN_POINT('',(-95.,-120.,-65.));
#30402=CARTESIAN_POINT('Origin',(-40.0000000000001,-120.,-265.));
#30403=CARTESIAN_POINT('',(-40.0000000000001,-115.,-265.));
#30404=CARTESIAN_POINT('',(-40.0000000000001,-115.,-265.));
#30405=CARTESIAN_POINT('',(-40.0000000000001,-120.,-265.));
#30406=CARTESIAN_POINT('',(-40.0000000000001,-120.,-265.));
#30407=CARTESIAN_POINT('',(-40.0000000000001,-120.,-265.));
#30408=CARTESIAN_POINT('Origin',(-40.0000000000001,-120.,-189.23552392847));
#30409=CARTESIAN_POINT('',(-40.0000000000001,-115.,-189.23552392847));
#30410=CARTESIAN_POINT('',(-40.0000000000001,-115.,-189.23552392847));
#30411=CARTESIAN_POINT('',(-40.0000000000001,-120.,-189.23552392847));
#30412=CARTESIAN_POINT('',(-40.0000000000001,-120.,-189.23552392847));
#30413=CARTESIAN_POINT('',(-40.0000000000001,-120.,-189.23552392847));
#30414=CARTESIAN_POINT('Origin',(39.9999999999999,-120.,-189.23552392847));
#30415=CARTESIAN_POINT('',(39.9999999999999,-115.,-189.23552392847));
#30416=CARTESIAN_POINT('',(39.9999999999999,-115.,-189.23552392847));
#30417=CARTESIAN_POINT('',(39.9999999999999,-120.,-189.23552392847));
#30418=CARTESIAN_POINT('',(39.9999999999999,-120.,-189.23552392847));
#30419=CARTESIAN_POINT('',(39.9999999999999,-120.,-189.23552392847));
#30420=CARTESIAN_POINT('Origin',(39.9999999999999,-120.,-265.));
#30421=CARTESIAN_POINT('',(39.9999999999999,-115.,-265.));
#30422=CARTESIAN_POINT('',(39.9999999999999,-115.,-265.));
#30423=CARTESIAN_POINT('',(39.9999999999999,-120.,-265.));
#30424=CARTESIAN_POINT('',(39.9999999999999,-120.,-265.));
#30425=CARTESIAN_POINT('',(39.9999999999999,-120.,-265.));
#30426=CARTESIAN_POINT('Origin',(95.,-120.,-265.));
#30427=CARTESIAN_POINT('',(95.,-115.,-265.));
#30428=CARTESIAN_POINT('',(95.,-120.,-265.));
#30429=CARTESIAN_POINT('Origin',(0.,-120.,0.));
#30430=CARTESIAN_POINT('Origin',(0.,-115.,0.));
#30431=CARTESIAN_POINT('',(100.,-115.,-55.9088729914395));
#30432=CARTESIAN_POINT('',(100.,-115.,-55.9088729914395));
#30433=CARTESIAN_POINT('',(100.,-115.,-265.));
#30434=CARTESIAN_POINT('',(100.,-115.,-55.9088729914395));
#30435=CARTESIAN_POINT('',(100.,-115.,-265.));
#30436=CARTESIAN_POINT('',(-100.,-115.,-265.));
#30437=CARTESIAN_POINT('',(-100.,-115.,-265.));
#30438=CARTESIAN_POINT('',(-100.,-115.,-55.9088729914395));
#30439=CARTESIAN_POINT('',(-100.,-115.,-55.9088729914395));
#30440=CARTESIAN_POINT('',(-100.,-115.,-55.9088729914395));
#30441=CARTESIAN_POINT('Origin',(100.,-284.055947712418,-511.630980392157));
#30442=CARTESIAN_POINT('',(100.,-284.055947712418,-511.630980392157));
#30443=CARTESIAN_POINT('',(100.,-284.055947712418,-511.630980392157));
#30444=CARTESIAN_POINT('',(100.,-284.055947712418,-511.630980392157));
#30445=CARTESIAN_POINT('Origin',(100.,-250.,-55.9088729914395));
#30446=CARTESIAN_POINT('',(100.,-250.,-55.9088729914395));
#30447=CARTESIAN_POINT('',(100.,-250.,-55.9088729914395));
#30448=CARTESIAN_POINT('',(100.,-250.,-55.9088729914395));
#30449=CARTESIAN_POINT('Origin',(100.,-250.,-55.9088729914395));
#30450=CARTESIAN_POINT('',(-581.975310925584,-250.,-444.538560851304));
#30451=CARTESIAN_POINT('',(-100.,-250.,-55.9088729914395));
#30452=CARTESIAN_POINT('',(-100.,-250.,-55.9088729914395));
#30453=CARTESIAN_POINT('',(-100.,-250.,42.3824489701997));
#30454=CARTESIAN_POINT('',(-100.,-250.,-55.9088729914395));
#30455=CARTESIAN_POINT('',(100.,-250.,42.3824489701997));
#30456=CARTESIAN_POINT('',(100.,-250.,42.3824489701997));
#30457=CARTESIAN_POINT('',(100.,-250.,-55.9088729914395));
#30458=CARTESIAN_POINT('Origin',(100.,-250.,42.3824489701997));
#30459=CARTESIAN_POINT('',(-100.,-391.404841890133,42.3824489701997));
#30460=CARTESIAN_POINT('',(-100.,-250.,42.3824489701997));
#30461=CARTESIAN_POINT('',(-100.,-391.404841890133,42.3824489701997));
#30462=CARTESIAN_POINT('',(-581.975310925585,-257.272114237069,42.3824489701997));
#30463=CARTESIAN_POINT('',(100.,-391.404841890133,42.3824489701997));
#30464=CARTESIAN_POINT('',(100.,-391.404841890133,42.3824489701997));
#30465=CARTESIAN_POINT('',(100.,-250.,42.3824489701997));
#30466=CARTESIAN_POINT('Origin',(100.,-391.404841890133,42.3824489701997));
#30467=CARTESIAN_POINT('',(100.,-391.404841890133,-511.630980392157));
#30468=CARTESIAN_POINT('',(100.,-391.404841890133,-511.630980392157));
#30469=CARTESIAN_POINT('',(100.,-391.404841890133,42.3824489701997));
#30470=CARTESIAN_POINT('Origin',(100.,-391.404841890133,-511.630980392157));
#30471=CARTESIAN_POINT('',(100.,-391.404841890133,-511.630980392157));
#30472=CARTESIAN_POINT('Origin',(100.,0.,1.13850834946031E-14));
#30473=CARTESIAN_POINT('Origin',(-100.,-284.055947712418,-511.630980392157));
#30474=CARTESIAN_POINT('',(-100.,-284.055947712418,-511.630980392157));
#30475=CARTESIAN_POINT('',(-100.,-284.055947712418,-511.630980392157));
#30476=CARTESIAN_POINT('',(-100.,-284.055947712418,-511.630980392157));
#30477=CARTESIAN_POINT('Origin',(-100.,-391.404841890133,-511.630980392157));
#30478=CARTESIAN_POINT('',(-100.,-391.404841890133,-511.630980392157));
#30479=CARTESIAN_POINT('',(-100.,-391.404841890133,-511.630980392157));
#30480=CARTESIAN_POINT('',(-100.,-391.404841890133,-511.630980392157));
#30481=CARTESIAN_POINT('Origin',(-100.,-391.404841890133,42.3824489701997));
#30482=CARTESIAN_POINT('',(-100.,-391.404841890133,42.3824489701997));
#30483=CARTESIAN_POINT('Origin',(-100.,-250.,-55.9088729914395));
#30484=CARTESIAN_POINT('',(-100.,-250.,-55.9088729914395));
#30485=CARTESIAN_POINT('Origin',(-100.,0.,1.13850834946031E-14));
#30486=CARTESIAN_POINT('Origin',(-581.975310925585,-257.272114237069,42.3824489701997));
#30487=CARTESIAN_POINT('',(-581.975310925584,-257.272114237069,-444.538560851304));
#30488=CARTESIAN_POINT('Origin',(-581.975310925584,-250.,-444.538560851304));
#39946=UNCERTAINTY_MEASURE_WITH_UNIT(LENGTH_MEASURE(0.01),#39960,
'DISTANCE_ACCURACY_VALUE',
'Maximum model space distance between geometric entities at asserted c
onnectivities');
#39950=UNCERTAINTY_MEASURE_WITH_UNIT(LENGTH_MEASURE(0.01),#39960,
'DISTANCE_ACCURACY_VALUE',
'Maximum model space distance between geometric entities at asserted c
onnectivities');
#39955=(
GEOMETRIC_REPRESENTATION_CONTEXT(3)
GLOBAL_UNCERTAINTY_ASSIGNED_CONTEXT((#39946))
GLOBAL_UNIT_ASSIGNED_CONTEXT((#39960,#39962,#39963))
REPRESENTATION_CONTEXT('','3D')
);
#39959=(
GEOMETRIC_REPRESENTATION_CONTEXT(3)
GLOBAL_UNCERTAINTY_ASSIGNED_CONTEXT((#39950))
GLOBAL_UNIT_ASSIGNED_CONTEXT((#39960,#39962,#39963))
REPRESENTATION_CONTEXT('','3D')
);
#39960=(
LENGTH_UNIT()
NAMED_UNIT(*)
SI_UNIT(.MILLI.,.METRE.)
);
#39962=(
NAMED_UNIT(*)
PLANE_ANGLE_UNIT()
SI_UNIT($,.RADIAN.)
);
#39963=(
NAMED_UNIT(*)
SI_UNIT($,.STERADIAN.)
SOLID_ANGLE_UNIT()
);
#39968=SHAPE_DEFINITION_REPRESENTATION(#39976,#40005);
#39976=PRODUCT_DEFINITION_SHAPE('',$,#40014);
#40005=SHAPE_REPRESENTATION('',(#18752),#39955);
#40009=PRODUCT_DEFINITION_CONTEXT('part definition',#40035,'design');
#40014=PRODUCT_DEFINITION('Motor Base','Motor Base',#40022,#40009);
#40022=PRODUCT_DEFINITION_FORMATION('',$,#40041);
#40035=APPLICATION_CONTEXT(
'Core Data for Automotive Mechanical Design Process');
#40036=PRODUCT_CONTEXT('part definition',#40035,'mechanical');
#40041=PRODUCT('Motor Base','Motor Base',$,(#40036));
#40046=PRESENTATION_STYLE_ASSIGNMENT((#40048));
#40048=SURFACE_STYLE_USAGE(.BOTH.,#40050);
#40050=SURFACE_SIDE_STYLE('',(#40052));
#40052=SURFACE_STYLE_FILL_AREA(#40054);
#40054=FILL_AREA_STYLE('Opaque(202,209,238)',(#40056));
#40056=FILL_AREA_STYLE_COLOUR('Opaque(202,209,238)',#40058);
#40058=COLOUR_RGB('Opaque(202,209,238)', 0.66274510, 0.83137255, 0.94901961);
ENDSEC;
END-ISO-10303-21;
